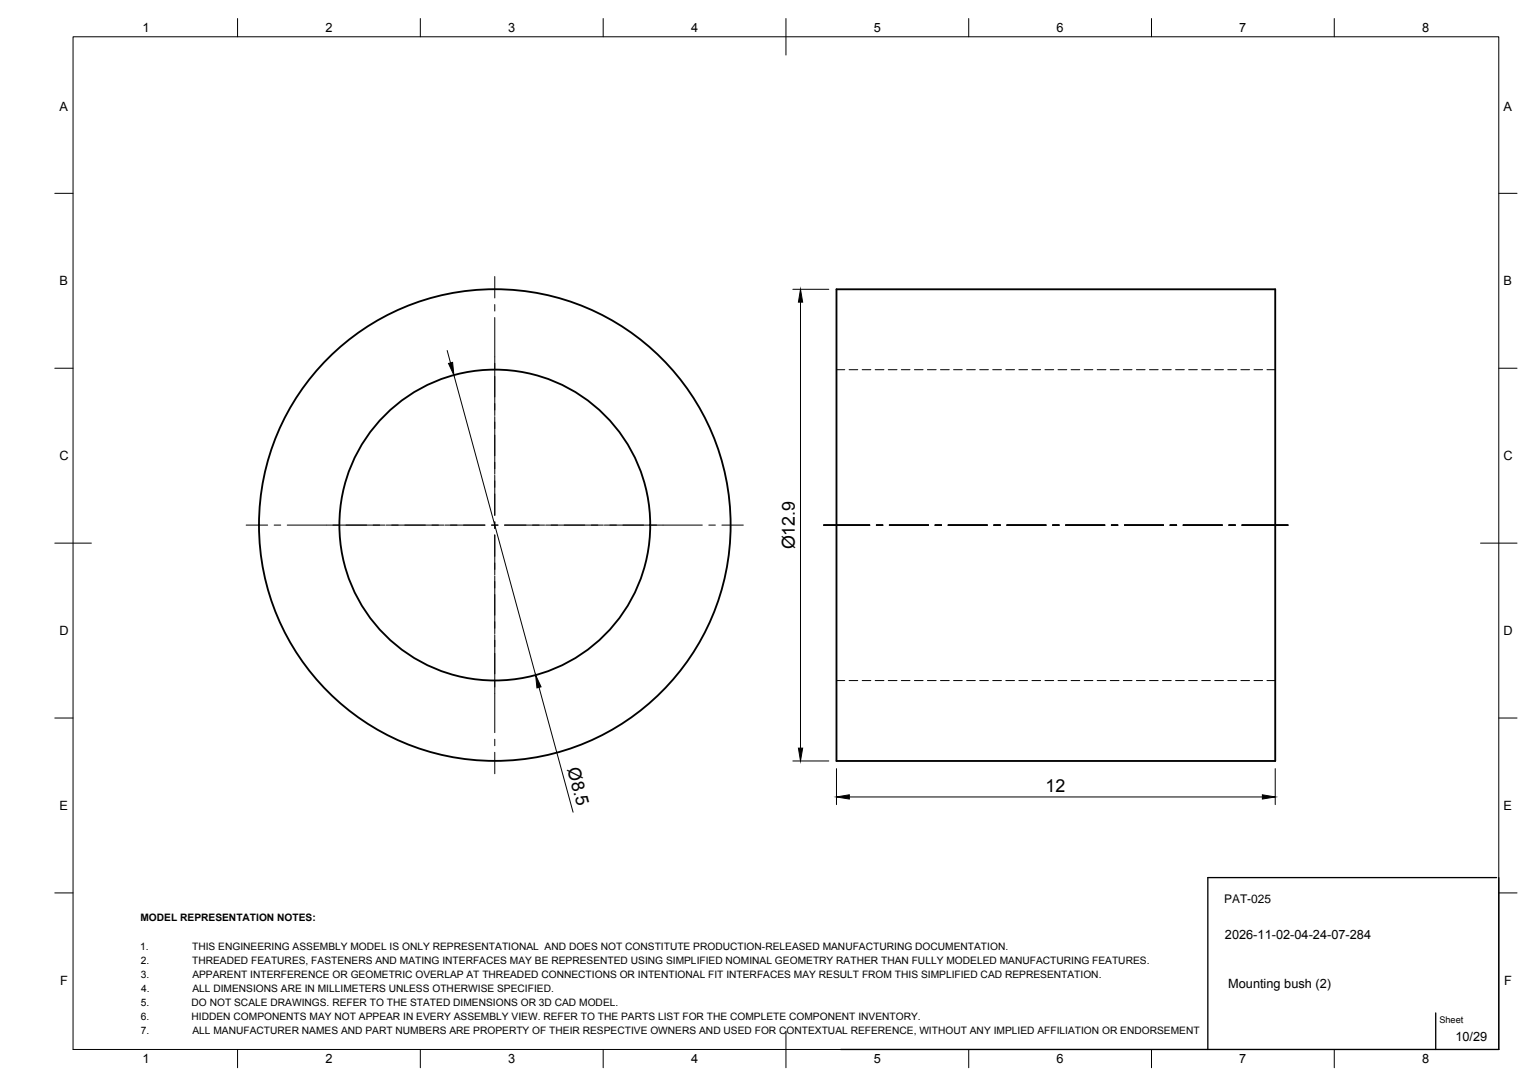
ISO-10303-21;
HEADER;
/* Generated by software containing ST-Developer
 * from STEP Tools, Inc. (www.steptools.com) 
 */

FILE_DESCRIPTION(
/* description */ ('Counter shaft with two pulleys and keyed hub'),
/* implementation_level */ '2;1');

FILE_NAME(
/* name */ 'Mounting bush (2).step',
/* time_stamp */ '2026-10-27T10:46:10-07:00',
/* author */ (''),
/* organization */ (''),
/* preprocessor_version */ 'ST-DEVELOPER v20.2',
/* originating_system */ 'Autodesk Translation Framework v15.17.0.0',
/* authorisation */ '');

FILE_SCHEMA (('AUTOMOTIVE_DESIGN { 1 0 10303 214 3 1 1 }'));
ENDSEC;

DATA;
#10=MECHANICAL_DESIGN_GEOMETRIC_PRESENTATION_REPRESENTATION('',(#295),#10821);
#245=SHAPE_REPRESENTATION_RELATIONSHIP('SRR','None',#10931,#270);
#270=ADVANCED_BREP_SHAPE_REPRESENTATION('',(#321),#10799);
#295=STYLED_ITEM('',(#11128),#321);
#321=MANIFOLD_SOLID_BREP('Body1',#5578);
#352=FACE_BOUND('',#947,.T.);
#353=FACE_BOUND('',#949,.T.);
#453=PLANE('',#5937);
#454=PLANE('',#5938);
#618=FACE_OUTER_BOUND('',#944,.T.);
#619=FACE_OUTER_BOUND('',#945,.T.);
#620=FACE_OUTER_BOUND('',#946,.T.);
#621=FACE_OUTER_BOUND('',#948,.T.);
#944=EDGE_LOOP('',(#3749,#3750,#3751,#3752));
#945=EDGE_LOOP('',(#3753,#3754,#3755,#3756));
#946=EDGE_LOOP('',(#3757));
#947=EDGE_LOOP('',(#3758));
#948=EDGE_LOOP('',(#3759));
#949=EDGE_LOOP('',(#3760));
#1351=LINE('',#8454,#1740);
#1352=LINE('',#8460,#1741);
#1740=VECTOR('',#6715,0.425);
#1741=VECTOR('',#6722,0.645);
#2101=CIRCLE('',#5932,0.425);
#2102=CIRCLE('',#5933,0.425);
#2103=CIRCLE('',#5935,0.645);
#2104=CIRCLE('',#5936,0.645);
#2424=VERTEX_POINT('',#8451);
#2425=VERTEX_POINT('',#8453);
#2426=VERTEX_POINT('',#8457);
#2427=VERTEX_POINT('',#8459);
#2947=EDGE_CURVE('',#2424,#2424,#2101,.T.);
#2948=EDGE_CURVE('',#2424,#2425,#1351,.T.);
#2949=EDGE_CURVE('',#2425,#2425,#2102,.T.);
#2950=EDGE_CURVE('',#2426,#2426,#2103,.T.);
#2951=EDGE_CURVE('',#2426,#2427,#1352,.T.);
#2952=EDGE_CURVE('',#2427,#2427,#2104,.T.);
#3749=ORIENTED_EDGE('',*,*,#2947,.F.);
#3750=ORIENTED_EDGE('',*,*,#2948,.T.);
#3751=ORIENTED_EDGE('',*,*,#2949,.T.);
#3752=ORIENTED_EDGE('',*,*,#2948,.F.);
#3753=ORIENTED_EDGE('',*,*,#2950,.F.);
#3754=ORIENTED_EDGE('',*,*,#2951,.T.);
#3755=ORIENTED_EDGE('',*,*,#2952,.T.);
#3756=ORIENTED_EDGE('',*,*,#2951,.F.);
#3757=ORIENTED_EDGE('',*,*,#2950,.T.);
#3758=ORIENTED_EDGE('',*,*,#2947,.T.);
#3759=ORIENTED_EDGE('',*,*,#2952,.F.);
#3760=ORIENTED_EDGE('',*,*,#2949,.F.);
#5121=CYLINDRICAL_SURFACE('',#5931,0.425);
#5122=CYLINDRICAL_SURFACE('',#5934,0.645);
#5289=ADVANCED_FACE('',(#618),#5121,.F.);
#5290=ADVANCED_FACE('',(#619),#5122,.T.);
#5291=ADVANCED_FACE('',(#620,#352),#453,.T.);
#5292=ADVANCED_FACE('',(#621,#353),#454,.F.);
#5578=CLOSED_SHELL('',(#5289,#5290,#5291,#5292));
#5930=AXIS2_PLACEMENT_3D('',#8449,#6709,#6710);
#5931=AXIS2_PLACEMENT_3D('',#8450,#6711,#6712);
#5932=AXIS2_PLACEMENT_3D('',#8452,#6713,#6714);
#5933=AXIS2_PLACEMENT_3D('',#8455,#6716,#6717);
#5934=AXIS2_PLACEMENT_3D('',#8456,#6718,#6719);
#5935=AXIS2_PLACEMENT_3D('',#8458,#6720,#6721);
#5936=AXIS2_PLACEMENT_3D('',#8461,#6723,#6724);
#5937=AXIS2_PLACEMENT_3D('',#8462,#6725,#6726);
#5938=AXIS2_PLACEMENT_3D('',#8463,#6727,#6728);
#6709=DIRECTION('axis',(0.,0.,1.));
#6710=DIRECTION('refdir',(1.,0.,0.));
#6711=DIRECTION('center_axis',(0.,0.,1.));
#6712=DIRECTION('ref_axis',(1.,0.,0.));
#6713=DIRECTION('center_axis',(0.,0.,-1.));
#6714=DIRECTION('ref_axis',(1.,0.,0.));
#6715=DIRECTION('',(0.,0.,-1.));
#6716=DIRECTION('center_axis',(0.,0.,-1.));
#6717=DIRECTION('ref_axis',(1.,0.,0.));
#6718=DIRECTION('center_axis',(0.,0.,1.));
#6719=DIRECTION('ref_axis',(1.,0.,0.));
#6720=DIRECTION('center_axis',(0.,0.,1.));
#6721=DIRECTION('ref_axis',(1.,0.,0.));
#6722=DIRECTION('',(0.,0.,-1.));
#6723=DIRECTION('center_axis',(0.,0.,1.));
#6724=DIRECTION('ref_axis',(1.,0.,0.));
#6725=DIRECTION('center_axis',(0.,0.,1.));
#6726=DIRECTION('ref_axis',(1.,0.,0.));
#6727=DIRECTION('center_axis',(0.,0.,1.));
#6728=DIRECTION('ref_axis',(1.,0.,0.));
#8449=CARTESIAN_POINT('',(0.,0.,0.));
#8450=CARTESIAN_POINT('Origin',(-4.75,20.,1.2));
#8451=CARTESIAN_POINT('',(-5.175,20.,2.4));
#8452=CARTESIAN_POINT('Origin',(-4.75,20.,2.4));
#8453=CARTESIAN_POINT('',(-5.175,20.,1.2));
#8454=CARTESIAN_POINT('',(-5.175,20.,1.2));
#8455=CARTESIAN_POINT('Origin',(-4.75,20.,1.2));
#8456=CARTESIAN_POINT('Origin',(-4.75,20.,1.2));
#8457=CARTESIAN_POINT('',(-5.395,20.,2.4));
#8458=CARTESIAN_POINT('Origin',(-4.75,20.,2.4));
#8459=CARTESIAN_POINT('',(-5.395,20.,1.2));
#8460=CARTESIAN_POINT('',(-5.395,20.,1.2));
#8461=CARTESIAN_POINT('Origin',(-4.75,20.,1.2));
#8462=CARTESIAN_POINT('Origin',(-4.75,20.,2.4));
#8463=CARTESIAN_POINT('Origin',(-4.75,20.,1.2));
#10769=UNCERTAINTY_MEASURE_WITH_UNIT(LENGTH_MEASURE(0.001),#10822,
'DISTANCE_ACCURACY_VALUE',
'Maximum model space distance between geometric entities at asserted c
onnectivities');
#10791=UNCERTAINTY_MEASURE_WITH_UNIT(LENGTH_MEASURE(0.001),#10822,
'DISTANCE_ACCURACY_VALUE',
'Maximum model space distance between geometric entities at asserted c
onnectivities');
#10799=(
GEOMETRIC_REPRESENTATION_CONTEXT(3)
GLOBAL_UNCERTAINTY_ASSIGNED_CONTEXT((#10769))
GLOBAL_UNIT_ASSIGNED_CONTEXT((#10822,#10824,#10825))
REPRESENTATION_CONTEXT('','3D')
);
#10821=(
GEOMETRIC_REPRESENTATION_CONTEXT(3)
GLOBAL_UNCERTAINTY_ASSIGNED_CONTEXT((#10791))
GLOBAL_UNIT_ASSIGNED_CONTEXT((#10822,#10824,#10825))
REPRESENTATION_CONTEXT('','3D')
);
#10822=(
LENGTH_UNIT()
NAMED_UNIT(*)
SI_UNIT(.CENTI.,.METRE.)
);
#10824=(
NAMED_UNIT(*)
PLANE_ANGLE_UNIT()
SI_UNIT($,.RADIAN.)
);
#10825=(
NAMED_UNIT(*)
SI_UNIT($,.STERADIAN.)
SOLID_ANGLE_UNIT()
);
#10833=SHAPE_DEFINITION_REPRESENTATION(#10862,#10931);
#10862=PRODUCT_DEFINITION_SHAPE('',$,#10961);
#10931=SHAPE_REPRESENTATION('',(#5930),#10799);
#10953=PRODUCT_DEFINITION_CONTEXT('part definition',#11042,'design');
#10961=PRODUCT_DEFINITION('Mounting bush (2)','Mounting bush (2)',#10990,
#10953);
#10990=PRODUCT_DEFINITION_FORMATION('',$,#11051);
#11042=APPLICATION_CONTEXT(
'Core Data for Automotive Mechanical Design Process');
#11043=PRODUCT_CONTEXT('part definition',#11042,'mechanical');
#11051=PRODUCT('Mounting bush (2)','Mounting bush (2)','Mounting bush (2)',(#11043));
#11122=COLOUR_RGB('Sky Blue',0.24,0.69,0.87);
#11123=FILL_AREA_STYLE_COLOUR('',#11122);
#11124=FILL_AREA_STYLE('',(#11123));
#11125=SURFACE_STYLE_FILL_AREA(#11124);
#11126=SURFACE_SIDE_STYLE('',(#11125));
#11127=SURFACE_STYLE_USAGE(.BOTH.,#11126);
#11128=PRESENTATION_STYLE_ASSIGNMENT((#11127));
ENDSEC;
END-ISO-10303-21;
